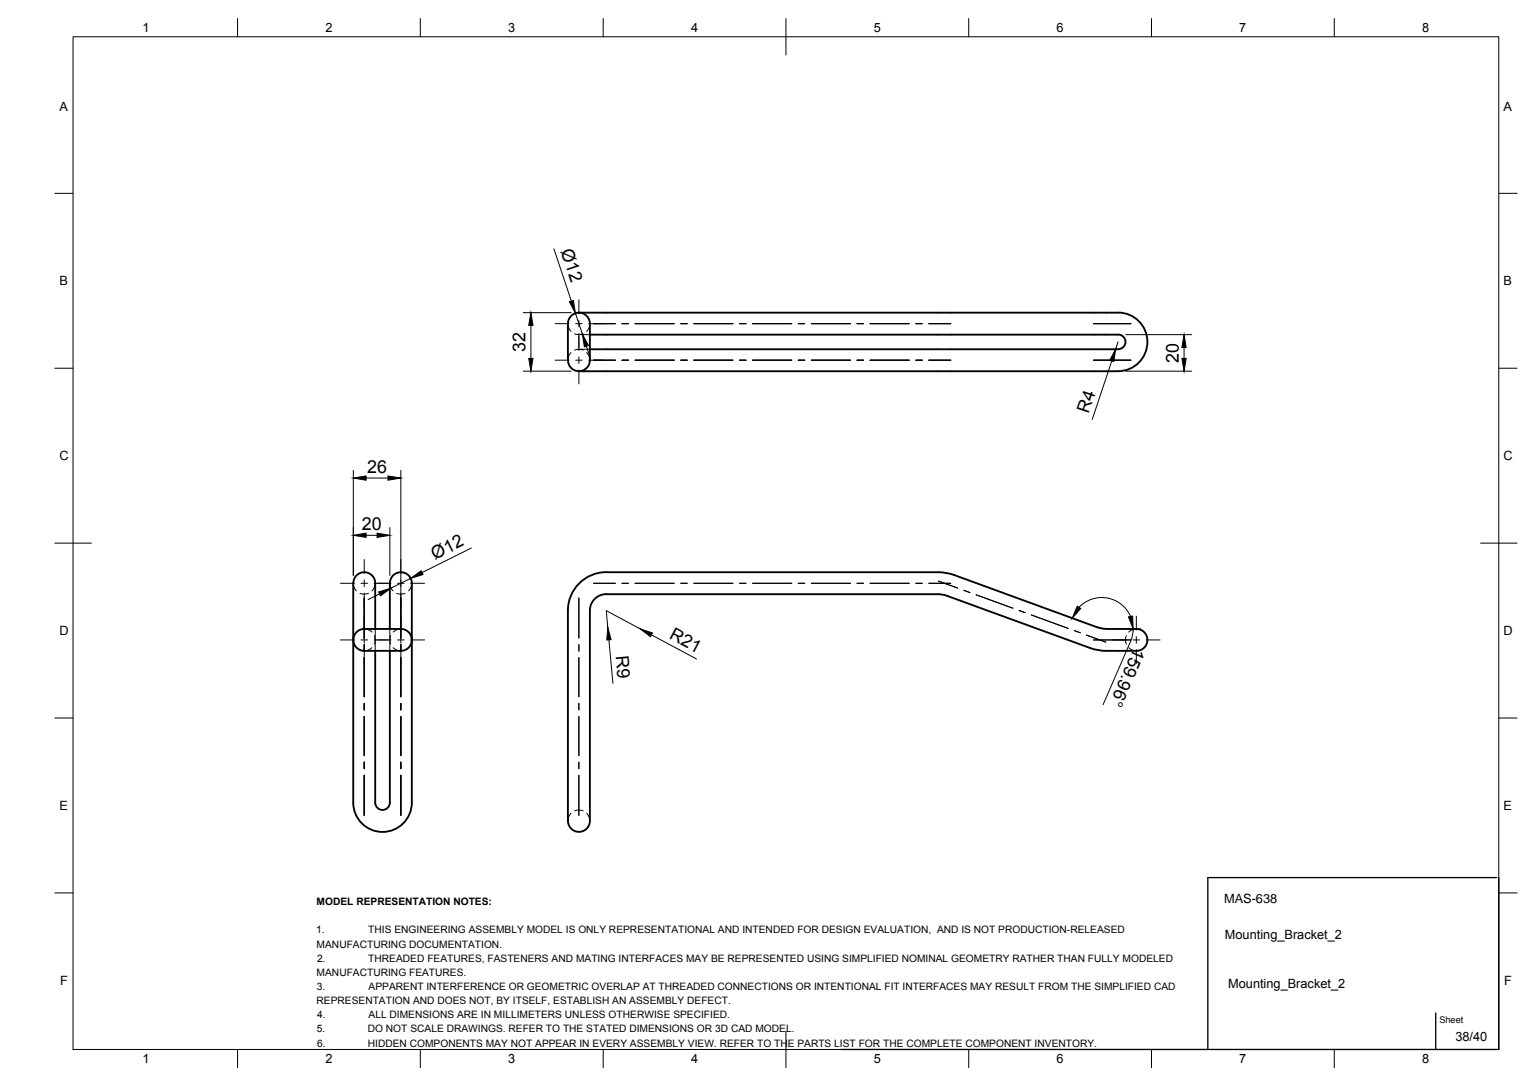
ISO-10303-21;
HEADER;
FILE_DESCRIPTION((''),'2;1');
FILE_NAME('Mounting_Bracket_2.step','2026-10-09T12:00:21-07:00',(''),(''),'','','');
FILE_SCHEMA (('AUTOMOTIVE_DESIGN { 1 0 10303 214 3 1 1 }'));
ENDSEC;
DATA;
#10=MECHANICAL_DESIGN_GEOMETRIC_PRESENTATION_REPRESENTATION('',(#433),#10334);
#168=CYLINDRICAL_SURFACE('',#4326,0.600000000000001) ;
#169=CYLINDRICAL_SURFACE('',#4327,0.600000000000001) ;
#170=CYLINDRICAL_SURFACE('',#4328,0.599999999999996) ;
#171=CYLINDRICAL_SURFACE('',#4329,0.600000000000001) ;
#172=CYLINDRICAL_SURFACE('',#4330,0.600000000000001) ;
#173=CYLINDRICAL_SURFACE('',#4331,0.600000000000001) ;
#174=CYLINDRICAL_SURFACE('',#4332,0.599999999999996) ;
#175=CYLINDRICAL_SURFACE('',#4333,0.600000000000001) ;
#361=SHAPE_REPRESENTATION_RELATIONSHIP('SRR','None',#10479,#393) ;
#393=ADVANCED_BREP_SHAPE_REPRESENTATION('',(#465),#10331) ;
#433=STYLED_ITEM('',(#10631),#465) ;
#465=MANIFOLD_SOLID_BREP('Body1',#3587) ;
#666=LINE('',#10068,#824) ;
#667=LINE('',#10070,#825) ;
#668=LINE('',#10072,#826) ;
#669=LINE('',#10074,#827) ;
#670=LINE('',#10076,#828) ;
#671=LINE('',#10078,#829) ;
#672=LINE('',#10080,#830) ;
#673=LINE('',#10082,#831) ;
#824=VECTOR('',#5346,0.600000000000001) ;
#825=VECTOR('',#5349,0.600000000000001) ;
#826=VECTOR('',#5352,0.599999999999996) ;
#827=VECTOR('',#5355,0.600000000000001) ;
#828=VECTOR('',#5358,0.600000000000001) ;
#829=VECTOR('',#5361,0.600000000000001) ;
#830=VECTOR('',#5364,0.599999999999996) ;
#831=VECTOR('',#5367,0.600000000000001) ;
#1002=FACE_OUTER_BOUND('',#1210,.T.) ;
#1003=FACE_OUTER_BOUND('',#1211,.T.) ;
#1004=FACE_OUTER_BOUND('',#1212,.T.) ;
#1005=FACE_OUTER_BOUND('',#1213,.T.) ;
#1006=FACE_OUTER_BOUND('',#1214,.T.) ;
#1007=FACE_OUTER_BOUND('',#1215,.T.) ;
#1008=FACE_OUTER_BOUND('',#1216,.T.) ;
#1009=FACE_OUTER_BOUND('',#1217,.T.) ;
#1010=FACE_OUTER_BOUND('',#1218,.T.) ;
#1011=FACE_OUTER_BOUND('',#1219,.T.) ;
#1012=FACE_OUTER_BOUND('',#1220,.T.) ;
#1013=FACE_OUTER_BOUND('',#1221,.T.) ;
#1014=FACE_OUTER_BOUND('',#1222,.T.) ;
#1015=FACE_OUTER_BOUND('',#1223,.T.) ;
#1016=FACE_OUTER_BOUND('',#1224,.T.) ;
#1017=FACE_OUTER_BOUND('',#1225,.T.) ;
#1210=EDGE_LOOP('',(#3049,#3050,#3051,#3052,#3053)) ;
#1211=EDGE_LOOP('',(#3054,#3055,#3056,#3057)) ;
#1212=EDGE_LOOP('',(#3058,#3059,#3060,#3061,#3062,#3063)) ;
#1213=EDGE_LOOP('',(#3064,#3065,#3066,#3067,#3068,#3069)) ;
#1214=EDGE_LOOP('',(#3070,#3071,#3072,#3073,#3074,#3075)) ;
#1215=EDGE_LOOP('',(#3076,#3077,#3078,#3079,#3080)) ;
#1216=EDGE_LOOP('',(#3081,#3082,#3083,#3084)) ;
#1217=EDGE_LOOP('',(#3085,#3086,#3087,#3088,#3089,#3090)) ;
#1218=EDGE_LOOP('',(#3091,#3092,#3093,#3094,#3095,#3096)) ;
#1219=EDGE_LOOP('',(#3097,#3098,#3099,#3100)) ;
#1220=EDGE_LOOP('',(#3101,#3102,#3103,#3104,#3105)) ;
#1221=EDGE_LOOP('',(#3106,#3107,#3108,#3109,#3110,#3111)) ;
#1222=EDGE_LOOP('',(#3112,#3113,#3114,#3115,#3116,#3117)) ;
#1223=EDGE_LOOP('',(#3118,#3119,#3120,#3121)) ;
#1224=EDGE_LOOP('',(#3122,#3123,#3124,#3125,#3126)) ;
#1225=EDGE_LOOP('',(#3127,#3128,#3129,#3130,#3131,#3132)) ;
#1397=CIRCLE('',#4285,0.600000000000001) ;
#1398=CIRCLE('',#4286,0.900000000000006) ;
#1399=CIRCLE('',#4287,0.600000000000001) ;
#1400=CIRCLE('',#4288,0.600000000000001) ;
#1401=CIRCLE('',#4290,0.600000000000001) ;
#1402=CIRCLE('',#4291,1.40000000000001) ;
#1403=CIRCLE('',#4292,0.600000000000001) ;
#1404=CIRCLE('',#4294,0.600000000000001) ;
#1405=CIRCLE('',#4295,0.600000000000001) ;
#1406=CIRCLE('',#4296,1.40000000000001) ;
#1407=CIRCLE('',#4297,0.600000000000001) ;
#1408=CIRCLE('',#4298,0.600000000000001) ;
#1409=CIRCLE('',#4300,0.600000000000001) ;
#1410=CIRCLE('',#4301,0.399999999999999) ;
#1411=CIRCLE('',#4302,0.600000000000001) ;
#1412=CIRCLE('',#4303,0.600000000000001) ;
#1413=CIRCLE('',#4304,0.600000000000001) ;
#1414=CIRCLE('',#4306,0.600000000000001) ;
#1415=CIRCLE('',#4307,0.600000000000001) ;
#1416=CIRCLE('',#4308,0.400000000000002) ;
#1417=CIRCLE('',#4309,0.600000000000001) ;
#1418=CIRCLE('',#4310,0.600000000000001) ;
#1419=CIRCLE('',#4312,0.600000000000001) ;
#1420=CIRCLE('',#4313,0.600000000000001) ;
#1421=CIRCLE('',#4314,0.900000000000006) ;
#1422=CIRCLE('',#4315,0.600000000000001) ;
#1423=CIRCLE('',#4317,0.600000000000001) ;
#1424=CIRCLE('',#4318,1.40000000000001) ;
#1425=CIRCLE('',#4319,0.600000000000001) ;
#1426=CIRCLE('',#4321,0.600000000000001) ;
#1427=CIRCLE('',#4322,0.600000000000001) ;
#1428=CIRCLE('',#4323,1.40000000000001) ;
#1429=CIRCLE('',#4324,0.600000000000001) ;
#1430=CIRCLE('',#4325,0.600000000000001) ;
#1732=VERTEX_POINT('',#10000) ;
#1733=VERTEX_POINT('',#10002) ;
#1734=VERTEX_POINT('',#10004) ;
#1735=VERTEX_POINT('',#10008) ;
#1736=VERTEX_POINT('',#10010) ;
#1737=VERTEX_POINT('',#10014) ;
#1738=VERTEX_POINT('',#10015) ;
#1739=VERTEX_POINT('',#10018) ;
#1740=VERTEX_POINT('',#10020) ;
#1741=VERTEX_POINT('',#10024) ;
#1742=VERTEX_POINT('',#10025) ;
#1743=VERTEX_POINT('',#10027) ;
#1744=VERTEX_POINT('',#10029) ;
#1745=VERTEX_POINT('',#10034) ;
#1746=VERTEX_POINT('',#10035) ;
#1747=VERTEX_POINT('',#10038) ;
#1748=VERTEX_POINT('',#10040) ;
#1749=VERTEX_POINT('',#10044) ;
#1750=VERTEX_POINT('',#10045) ;
#1751=VERTEX_POINT('',#10048) ;
#1752=VERTEX_POINT('',#10052) ;
#1753=VERTEX_POINT('',#10054) ;
#1754=VERTEX_POINT('',#10058) ;
#1755=VERTEX_POINT('',#10059) ;
#1756=VERTEX_POINT('',#10062) ;
#1757=VERTEX_POINT('',#10064) ;
#2181=EDGE_CURVE('',#1732,#1732,#1397,.T.) ;
#2182=EDGE_CURVE('',#1732,#1733,#1398,.T.) ;
#2183=EDGE_CURVE('',#1733,#1734,#1399,.T.) ;
#2184=EDGE_CURVE('',#1734,#1733,#1400,.T.) ;
#2185=EDGE_CURVE('',#1735,#1735,#1401,.T.) ;
#2186=EDGE_CURVE('',#1735,#1736,#1402,.T.) ;
#2187=EDGE_CURVE('',#1736,#1736,#1403,.T.) ;
#2188=EDGE_CURVE('',#1737,#1738,#1404,.T.) ;
#2189=EDGE_CURVE('',#1738,#1737,#1405,.T.) ;
#2190=EDGE_CURVE('',#1738,#1739,#1406,.T.) ;
#2191=EDGE_CURVE('',#1739,#1740,#1407,.T.) ;
#2192=EDGE_CURVE('',#1740,#1739,#1408,.T.) ;
#2193=EDGE_CURVE('',#1741,#1742,#1409,.T.) ;
#2194=EDGE_CURVE('',#1742,#1743,#1410,.T.) ;
#2195=EDGE_CURVE('',#1744,#1743,#1411,.T.) ;
#2196=EDGE_CURVE('',#1743,#1744,#1412,.T.) ;
#2197=EDGE_CURVE('',#1742,#1741,#1413,.T.) ;
#2198=EDGE_CURVE('',#1745,#1746,#1414,.T.) ;
#2199=EDGE_CURVE('',#1746,#1745,#1415,.T.) ;
#2200=EDGE_CURVE('',#1746,#1747,#1416,.T.) ;
#2201=EDGE_CURVE('',#1747,#1748,#1417,.T.) ;
#2202=EDGE_CURVE('',#1748,#1747,#1418,.T.) ;
#2203=EDGE_CURVE('',#1749,#1750,#1419,.T.) ;
#2204=EDGE_CURVE('',#1750,#1749,#1420,.T.) ;
#2205=EDGE_CURVE('',#1750,#1751,#1421,.T.) ;
#2206=EDGE_CURVE('',#1751,#1751,#1422,.T.) ;
#2207=EDGE_CURVE('',#1752,#1752,#1423,.T.) ;
#2208=EDGE_CURVE('',#1752,#1753,#1424,.T.) ;
#2209=EDGE_CURVE('',#1753,#1753,#1425,.T.) ;
#2210=EDGE_CURVE('',#1754,#1755,#1426,.T.) ;
#2211=EDGE_CURVE('',#1755,#1754,#1427,.T.) ;
#2212=EDGE_CURVE('',#1755,#1756,#1428,.T.) ;
#2213=EDGE_CURVE('',#1756,#1757,#1429,.T.) ;
#2214=EDGE_CURVE('',#1757,#1756,#1430,.T.) ;
#2215=EDGE_CURVE('',#1745,#1734,#666,.T.) ;
#2216=EDGE_CURVE('',#1732,#1736,#667,.T.) ;
#2217=EDGE_CURVE('',#1735,#1740,#668,.T.) ;
#2218=EDGE_CURVE('',#1737,#1741,#669,.T.) ;
#2219=EDGE_CURVE('',#1748,#1749,#670,.T.) ;
#2220=EDGE_CURVE('',#1751,#1752,#671,.T.) ;
#2221=EDGE_CURVE('',#1753,#1754,#672,.T.) ;
#2222=EDGE_CURVE('',#1757,#1744,#673,.T.) ;
#3049=ORIENTED_EDGE('',*,*,#2181,.F.) ;
#3050=ORIENTED_EDGE('',*,*,#2182,.T.) ;
#3051=ORIENTED_EDGE('',*,*,#2183,.T.) ;
#3052=ORIENTED_EDGE('',*,*,#2184,.T.) ;
#3053=ORIENTED_EDGE('',*,*,#2182,.F.) ;
#3054=ORIENTED_EDGE('',*,*,#2185,.F.) ;
#3055=ORIENTED_EDGE('',*,*,#2186,.T.) ;
#3056=ORIENTED_EDGE('',*,*,#2187,.T.) ;
#3057=ORIENTED_EDGE('',*,*,#2186,.F.) ;
#3058=ORIENTED_EDGE('',*,*,#2188,.F.) ;
#3059=ORIENTED_EDGE('',*,*,#2189,.F.) ;
#3060=ORIENTED_EDGE('',*,*,#2190,.T.) ;
#3061=ORIENTED_EDGE('',*,*,#2191,.T.) ;
#3062=ORIENTED_EDGE('',*,*,#2192,.T.) ;
#3063=ORIENTED_EDGE('',*,*,#2190,.F.) ;
#3064=ORIENTED_EDGE('',*,*,#2193,.T.) ;
#3065=ORIENTED_EDGE('',*,*,#2194,.T.) ;
#3066=ORIENTED_EDGE('',*,*,#2195,.F.) ;
#3067=ORIENTED_EDGE('',*,*,#2196,.F.) ;
#3068=ORIENTED_EDGE('',*,*,#2194,.F.) ;
#3069=ORIENTED_EDGE('',*,*,#2197,.T.) ;
#3070=ORIENTED_EDGE('',*,*,#2198,.F.) ;
#3071=ORIENTED_EDGE('',*,*,#2199,.F.) ;
#3072=ORIENTED_EDGE('',*,*,#2200,.T.) ;
#3073=ORIENTED_EDGE('',*,*,#2201,.T.) ;
#3074=ORIENTED_EDGE('',*,*,#2202,.T.) ;
#3075=ORIENTED_EDGE('',*,*,#2200,.F.) ;
#3076=ORIENTED_EDGE('',*,*,#2203,.F.) ;
#3077=ORIENTED_EDGE('',*,*,#2204,.F.) ;
#3078=ORIENTED_EDGE('',*,*,#2205,.T.) ;
#3079=ORIENTED_EDGE('',*,*,#2206,.T.) ;
#3080=ORIENTED_EDGE('',*,*,#2205,.F.) ;
#3081=ORIENTED_EDGE('',*,*,#2207,.F.) ;
#3082=ORIENTED_EDGE('',*,*,#2208,.T.) ;
#3083=ORIENTED_EDGE('',*,*,#2209,.T.) ;
#3084=ORIENTED_EDGE('',*,*,#2208,.F.) ;
#3085=ORIENTED_EDGE('',*,*,#2210,.F.) ;
#3086=ORIENTED_EDGE('',*,*,#2211,.F.) ;
#3087=ORIENTED_EDGE('',*,*,#2212,.T.) ;
#3088=ORIENTED_EDGE('',*,*,#2213,.T.) ;
#3089=ORIENTED_EDGE('',*,*,#2214,.T.) ;
#3090=ORIENTED_EDGE('',*,*,#2212,.F.) ;
#3091=ORIENTED_EDGE('',*,*,#2198,.T.) ;
#3092=ORIENTED_EDGE('',*,*,#2199,.T.) ;
#3093=ORIENTED_EDGE('',*,*,#2215,.T.) ;
#3094=ORIENTED_EDGE('',*,*,#2183,.F.) ;
#3095=ORIENTED_EDGE('',*,*,#2184,.F.) ;
#3096=ORIENTED_EDGE('',*,*,#2215,.F.) ;
#3097=ORIENTED_EDGE('',*,*,#2181,.T.) ;
#3098=ORIENTED_EDGE('',*,*,#2216,.T.) ;
#3099=ORIENTED_EDGE('',*,*,#2187,.F.) ;
#3100=ORIENTED_EDGE('',*,*,#2216,.F.) ;
#3101=ORIENTED_EDGE('',*,*,#2185,.T.) ;
#3102=ORIENTED_EDGE('',*,*,#2217,.T.) ;
#3103=ORIENTED_EDGE('',*,*,#2191,.F.) ;
#3104=ORIENTED_EDGE('',*,*,#2192,.F.) ;
#3105=ORIENTED_EDGE('',*,*,#2217,.F.) ;
#3106=ORIENTED_EDGE('',*,*,#2188,.T.) ;
#3107=ORIENTED_EDGE('',*,*,#2189,.T.) ;
#3108=ORIENTED_EDGE('',*,*,#2218,.T.) ;
#3109=ORIENTED_EDGE('',*,*,#2197,.F.) ;
#3110=ORIENTED_EDGE('',*,*,#2193,.F.) ;
#3111=ORIENTED_EDGE('',*,*,#2218,.F.) ;
#3112=ORIENTED_EDGE('',*,*,#2202,.F.) ;
#3113=ORIENTED_EDGE('',*,*,#2219,.T.) ;
#3114=ORIENTED_EDGE('',*,*,#2203,.T.) ;
#3115=ORIENTED_EDGE('',*,*,#2204,.T.) ;
#3116=ORIENTED_EDGE('',*,*,#2219,.F.) ;
#3117=ORIENTED_EDGE('',*,*,#2201,.F.) ;
#3118=ORIENTED_EDGE('',*,*,#2206,.F.) ;
#3119=ORIENTED_EDGE('',*,*,#2220,.T.) ;
#3120=ORIENTED_EDGE('',*,*,#2207,.T.) ;
#3121=ORIENTED_EDGE('',*,*,#2220,.F.) ;
#3122=ORIENTED_EDGE('',*,*,#2209,.F.) ;
#3123=ORIENTED_EDGE('',*,*,#2221,.T.) ;
#3124=ORIENTED_EDGE('',*,*,#2210,.T.) ;
#3125=ORIENTED_EDGE('',*,*,#2211,.T.) ;
#3126=ORIENTED_EDGE('',*,*,#2221,.F.) ;
#3127=ORIENTED_EDGE('',*,*,#2214,.F.) ;
#3128=ORIENTED_EDGE('',*,*,#2222,.T.) ;
#3129=ORIENTED_EDGE('',*,*,#2195,.T.) ;
#3130=ORIENTED_EDGE('',*,*,#2196,.T.) ;
#3131=ORIENTED_EDGE('',*,*,#2222,.F.) ;
#3132=ORIENTED_EDGE('',*,*,#2213,.F.) ;
#3335=TOROIDAL_SURFACE('',#4284,1.5,0.6) ;
#3336=TOROIDAL_SURFACE('',#4289,2.,0.6) ;
#3337=TOROIDAL_SURFACE('',#4293,2.,0.6) ;
#3338=TOROIDAL_SURFACE('',#4299,1.,0.6) ;
#3339=TOROIDAL_SURFACE('',#4305,1.,0.599999999999999) ;
#3340=TOROIDAL_SURFACE('',#4311,1.5,0.6) ;
#3341=TOROIDAL_SURFACE('',#4316,2.,0.6) ;
#3342=TOROIDAL_SURFACE('',#4320,2.,0.6) ;
#3510=ADVANCED_FACE('',(#1002),#3335,.T.) ;
#3511=ADVANCED_FACE('',(#1003),#3336,.T.) ;
#3512=ADVANCED_FACE('',(#1004),#3337,.T.) ;
#3513=ADVANCED_FACE('',(#1005),#3338,.T.) ;
#3514=ADVANCED_FACE('',(#1006),#3339,.T.) ;
#3515=ADVANCED_FACE('',(#1007),#3340,.T.) ;
#3516=ADVANCED_FACE('',(#1008),#3341,.T.) ;
#3517=ADVANCED_FACE('',(#1009),#3342,.T.) ;
#3518=ADVANCED_FACE('',(#1010),#168,.T.) ;
#3519=ADVANCED_FACE('',(#1011),#169,.T.) ;
#3520=ADVANCED_FACE('',(#1012),#170,.T.) ;
#3521=ADVANCED_FACE('',(#1013),#171,.T.) ;
#3522=ADVANCED_FACE('',(#1014),#172,.T.) ;
#3523=ADVANCED_FACE('',(#1015),#173,.T.) ;
#3524=ADVANCED_FACE('',(#1016),#174,.T.) ;
#3525=ADVANCED_FACE('',(#1017),#175,.T.) ;
#3587=CLOSED_SHELL('',(#3510,#3511,#3512,#3513,#3514,#3515,#3516,#3517,
#3518,#3519,#3520,#3521,#3522,#3523,#3524,#3525)) ;
#4283=AXIS2_PLACEMENT_3D('',#9998,#5258,#5259) ;
#4284=AXIS2_PLACEMENT_3D('',#9999,#5260,#5261) ;
#4285=AXIS2_PLACEMENT_3D('',#10001,#5262,#5263) ;
#4286=AXIS2_PLACEMENT_3D('',#10003,#5264,#5265) ;
#4287=AXIS2_PLACEMENT_3D('',#10005,#5266,#5267) ;
#4288=AXIS2_PLACEMENT_3D('',#10006,#5268,#5269) ;
#4289=AXIS2_PLACEMENT_3D('',#10007,#5270,#5271) ;
#4290=AXIS2_PLACEMENT_3D('',#10009,#5272,#5273) ;
#4291=AXIS2_PLACEMENT_3D('',#10011,#5274,#5275) ;
#4292=AXIS2_PLACEMENT_3D('',#10012,#5276,#5277) ;
#4293=AXIS2_PLACEMENT_3D('',#10013,#5278,#5279) ;
#4294=AXIS2_PLACEMENT_3D('',#10016,#5280,#5281) ;
#4295=AXIS2_PLACEMENT_3D('',#10017,#5282,#5283) ;
#4296=AXIS2_PLACEMENT_3D('',#10019,#5284,#5285) ;
#4297=AXIS2_PLACEMENT_3D('',#10021,#5286,#5287) ;
#4298=AXIS2_PLACEMENT_3D('',#10022,#5288,#5289) ;
#4299=AXIS2_PLACEMENT_3D('',#10023,#5290,#5291) ;
#4300=AXIS2_PLACEMENT_3D('',#10026,#5292,#5293) ;
#4301=AXIS2_PLACEMENT_3D('',#10028,#5294,#5295) ;
#4302=AXIS2_PLACEMENT_3D('',#10030,#5296,#5297) ;
#4303=AXIS2_PLACEMENT_3D('',#10031,#5298,#5299) ;
#4304=AXIS2_PLACEMENT_3D('',#10032,#5300,#5301) ;
#4305=AXIS2_PLACEMENT_3D('',#10033,#5302,#5303) ;
#4306=AXIS2_PLACEMENT_3D('',#10036,#5304,#5305) ;
#4307=AXIS2_PLACEMENT_3D('',#10037,#5306,#5307) ;
#4308=AXIS2_PLACEMENT_3D('',#10039,#5308,#5309) ;
#4309=AXIS2_PLACEMENT_3D('',#10041,#5310,#5311) ;
#4310=AXIS2_PLACEMENT_3D('',#10042,#5312,#5313) ;
#4311=AXIS2_PLACEMENT_3D('',#10043,#5314,#5315) ;
#4312=AXIS2_PLACEMENT_3D('',#10046,#5316,#5317) ;
#4313=AXIS2_PLACEMENT_3D('',#10047,#5318,#5319) ;
#4314=AXIS2_PLACEMENT_3D('',#10049,#5320,#5321) ;
#4315=AXIS2_PLACEMENT_3D('',#10050,#5322,#5323) ;
#4316=AXIS2_PLACEMENT_3D('',#10051,#5324,#5325) ;
#4317=AXIS2_PLACEMENT_3D('',#10053,#5326,#5327) ;
#4318=AXIS2_PLACEMENT_3D('',#10055,#5328,#5329) ;
#4319=AXIS2_PLACEMENT_3D('',#10056,#5330,#5331) ;
#4320=AXIS2_PLACEMENT_3D('',#10057,#5332,#5333) ;
#4321=AXIS2_PLACEMENT_3D('',#10060,#5334,#5335) ;
#4322=AXIS2_PLACEMENT_3D('',#10061,#5336,#5337) ;
#4323=AXIS2_PLACEMENT_3D('',#10063,#5338,#5339) ;
#4324=AXIS2_PLACEMENT_3D('',#10065,#5340,#5341) ;
#4325=AXIS2_PLACEMENT_3D('',#10066,#5342,#5343) ;
#4326=AXIS2_PLACEMENT_3D('',#10067,#5344,#5345) ;
#4327=AXIS2_PLACEMENT_3D('',#10069,#5347,#5348) ;
#4328=AXIS2_PLACEMENT_3D('',#10071,#5350,#5351) ;
#4329=AXIS2_PLACEMENT_3D('',#10073,#5353,#5354) ;
#4330=AXIS2_PLACEMENT_3D('',#10075,#5356,#5357) ;
#4331=AXIS2_PLACEMENT_3D('',#10077,#5359,#5360) ;
#4332=AXIS2_PLACEMENT_3D('',#10079,#5362,#5363) ;
#4333=AXIS2_PLACEMENT_3D('',#10081,#5365,#5366) ;
#5258=DIRECTION('axis',(0.,0.,1.)) ;
#5259=DIRECTION('refdir',(1.,0.,0.)) ;
#5260=DIRECTION('center_axis',(-1.,0.,-3.38946600347724E-15)) ;
#5261=DIRECTION('ref_axis',(3.38353683695287E-15,0.,-1.)) ;
#5262=DIRECTION('center_axis',(3.38946600347724E-15,0.,-1.)) ;
#5263=DIRECTION('ref_axis',(-1.,0.,-3.38946600347724E-15)) ;
#5264=DIRECTION('center_axis',(1.,0.,3.38946600347724E-15)) ;
#5265=DIRECTION('ref_axis',(3.38946600347724E-15,0.,-1.)) ;
#5266=DIRECTION('center_axis',(0.,1.,0.)) ;
#5267=DIRECTION('ref_axis',(-1.,0.,0.)) ;
#5268=DIRECTION('center_axis',(0.,1.,0.)) ;
#5269=DIRECTION('ref_axis',(-1.,0.,0.)) ;
#5270=DIRECTION('center_axis',(-1.,0.,-3.38946600347724E-15)) ;
#5271=DIRECTION('ref_axis',(4.09928501400059E-15,0.,-1.)) ;
#5272=DIRECTION('center_axis',(3.1843026467959E-15,-0.342630345100702,-0.93947030108257)) ;
#5273=DIRECTION('ref_axis',(-1.,-1.09103871477676E-15,-2.99155776632337E-15)) ;
#5274=DIRECTION('center_axis',(1.,0.,3.38946600347724E-15)) ;
#5275=DIRECTION('ref_axis',(3.38946600347724E-15,0.,-1.)) ;
#5276=DIRECTION('center_axis',(3.38946600347724E-15,0.,-1.)) ;
#5277=DIRECTION('ref_axis',(-1.,0.,-3.38946600347724E-15)) ;
#5278=DIRECTION('center_axis',(1.,0.,3.38946600347724E-15)) ;
#5279=DIRECTION('ref_axis',(-4.09928501400059E-15,0.,1.)) ;
#5280=DIRECTION('center_axis',(3.38946600347724E-15,0.,-1.)) ;
#5281=DIRECTION('ref_axis',(-1.,0.,-3.38946600347724E-15)) ;
#5282=DIRECTION('center_axis',(3.38946600347724E-15,0.,-1.)) ;
#5283=DIRECTION('ref_axis',(-1.,0.,-3.38946600347724E-15)) ;
#5284=DIRECTION('center_axis',(-1.,0.,-3.38946600347724E-15)) ;
#5285=DIRECTION('ref_axis',(-3.38946600347724E-15,0.,1.)) ;
#5286=DIRECTION('center_axis',(3.1843026467959E-15,-0.342630345100702,-0.93947030108257)) ;
#5287=DIRECTION('ref_axis',(-1.,-1.09103871477676E-15,-2.99155776632337E-15)) ;
#5288=DIRECTION('center_axis',(3.1843026467959E-15,-0.342630345100702,-0.93947030108257)) ;
#5289=DIRECTION('ref_axis',(-1.,-1.09103871477676E-15,-2.99155776632337E-15)) ;
#5290=DIRECTION('center_axis',(0.,-1.,0.)) ;
#5291=DIRECTION('ref_axis',(1.,0.,0.)) ;
#5292=DIRECTION('center_axis',(3.38946600347724E-15,0.,-1.)) ;
#5293=DIRECTION('ref_axis',(-1.,0.,-3.38946600347724E-15)) ;
#5294=DIRECTION('center_axis',(0.,1.,0.)) ;
#5295=DIRECTION('ref_axis',(1.,0.,0.)) ;
#5296=DIRECTION('center_axis',(-3.49148133884313E-15,0.,1.)) ;
#5297=DIRECTION('ref_axis',(1.,0.,3.49148133884313E-15)) ;
#5298=DIRECTION('center_axis',(-3.49148133884313E-15,0.,1.)) ;
#5299=DIRECTION('ref_axis',(1.,0.,3.49148133884313E-15)) ;
#5300=DIRECTION('center_axis',(3.38946600347724E-15,0.,-1.)) ;
#5301=DIRECTION('ref_axis',(-1.,0.,-3.38946600347724E-15)) ;
#5302=DIRECTION('center_axis',(-3.49148133884313E-15,0.,1.)) ;
#5303=DIRECTION('ref_axis',(1.,0.,0.)) ;
#5304=DIRECTION('center_axis',(0.,1.,0.)) ;
#5305=DIRECTION('ref_axis',(-1.,0.,0.)) ;
#5306=DIRECTION('center_axis',(0.,1.,0.)) ;
#5307=DIRECTION('ref_axis',(-1.,0.,0.)) ;
#5308=DIRECTION('center_axis',(3.49148133884313E-15,0.,-1.)) ;
#5309=DIRECTION('ref_axis',(1.,0.,3.49148133884313E-15)) ;
#5310=DIRECTION('center_axis',(0.,-1.,0.)) ;
#5311=DIRECTION('ref_axis',(1.,0.,0.)) ;
#5312=DIRECTION('center_axis',(0.,-1.,0.)) ;
#5313=DIRECTION('ref_axis',(1.,0.,0.)) ;
#5314=DIRECTION('center_axis',(1.,0.,3.49148133884313E-15)) ;
#5315=DIRECTION('ref_axis',(3.38353683695287E-15,0.,-1.)) ;
#5316=DIRECTION('center_axis',(0.,-1.,0.)) ;
#5317=DIRECTION('ref_axis',(1.,0.,0.)) ;
#5318=DIRECTION('center_axis',(0.,-1.,0.)) ;
#5319=DIRECTION('ref_axis',(1.,0.,0.)) ;
#5320=DIRECTION('center_axis',(-1.,0.,-3.49148133884313E-15)) ;
#5321=DIRECTION('ref_axis',(3.49148133884313E-15,0.,-1.)) ;
#5322=DIRECTION('center_axis',(-3.49148133884313E-15,0.,1.)) ;
#5323=DIRECTION('ref_axis',(1.,0.,3.49148133884313E-15)) ;
#5324=DIRECTION('center_axis',(1.,0.,3.49148133884313E-15)) ;
#5325=DIRECTION('ref_axis',(4.09928501400059E-15,0.,-1.)) ;
#5326=DIRECTION('center_axis',(-3.49148133884313E-15,0.,1.)) ;
#5327=DIRECTION('ref_axis',(1.,0.,3.49148133884313E-15)) ;
#5328=DIRECTION('center_axis',(-1.,0.,-3.49148133884313E-15)) ;
#5329=DIRECTION('ref_axis',(3.49148133884313E-15,0.,-1.)) ;
#5330=DIRECTION('center_axis',(-3.28014302462713E-15,0.342630345100702,
0.93947030108257)) ;
#5331=DIRECTION('ref_axis',(1.,1.12387653650765E-15,3.08159695494034E-15)) ;
#5332=DIRECTION('center_axis',(-1.,0.,-3.49148133884313E-15)) ;
#5333=DIRECTION('ref_axis',(-4.09928501400059E-15,0.,1.)) ;
#5334=DIRECTION('center_axis',(-3.28014302462713E-15,0.342630345100702,
0.93947030108257)) ;
#5335=DIRECTION('ref_axis',(1.,1.12387653650765E-15,3.08159695494034E-15)) ;
#5336=DIRECTION('center_axis',(-3.28014302462713E-15,0.342630345100702,
0.93947030108257)) ;
#5337=DIRECTION('ref_axis',(1.,1.12387653650765E-15,3.08159695494034E-15)) ;
#5338=DIRECTION('center_axis',(1.,0.,3.49148133884313E-15)) ;
#5339=DIRECTION('ref_axis',(-3.49148133884313E-15,0.,1.)) ;
#5340=DIRECTION('center_axis',(-3.49148133884313E-15,0.,1.)) ;
#5341=DIRECTION('ref_axis',(1.,0.,3.49148133884313E-15)) ;
#5342=DIRECTION('center_axis',(-3.49148133884313E-15,0.,1.)) ;
#5343=DIRECTION('ref_axis',(1.,0.,3.49148133884313E-15)) ;
#5344=DIRECTION('center_axis',(0.,-1.,0.)) ;
#5345=DIRECTION('ref_axis',(-1.,0.,0.)) ;
#5346=DIRECTION('',(0.,1.,0.)) ;
#5347=DIRECTION('center_axis',(-3.38946600347724E-15,1.91189112624469E-17,
1.)) ;
#5348=DIRECTION('ref_axis',(6.48028997475618E-32,1.,-1.91189112624469E-17)) ;
#5349=DIRECTION('',(3.38946600347724E-15,-1.91189112624469E-17,-1.)) ;
#5350=DIRECTION('center_axis',(-3.1843026467959E-15,0.342630345100702,0.93947030108257)) ;
#5351=DIRECTION('ref_axis',(1.13665102922496E-30,0.93947030108257,-0.342630345100702)) ;
#5352=DIRECTION('',(3.1843026467959E-15,-0.342630345100702,-0.93947030108257)) ;
#5353=DIRECTION('center_axis',(-3.38946600347724E-15,0.,1.)) ;
#5354=DIRECTION('ref_axis',(-1.,0.,-3.38946600347724E-15)) ;
#5355=DIRECTION('',(3.38946600347724E-15,0.,-1.)) ;
#5356=DIRECTION('center_axis',(0.,-1.,0.)) ;
#5357=DIRECTION('ref_axis',(1.,0.,0.)) ;
#5358=DIRECTION('',(0.,1.,0.)) ;
#5359=DIRECTION('center_axis',(-3.49148133884313E-15,1.91189112624469E-17,
1.)) ;
#5360=DIRECTION('ref_axis',(6.6753321891831E-32,1.,-1.91189112624469E-17)) ;
#5361=DIRECTION('',(3.49148133884313E-15,-1.91189112624469E-17,-1.)) ;
#5362=DIRECTION('center_axis',(-3.28014302462713E-15,0.342630345100702,
0.93947030108257)) ;
#5363=DIRECTION('ref_axis',(1.24553608015764E-30,0.93947030108257,-0.342630345100702)) ;
#5364=DIRECTION('',(3.28014302462713E-15,-0.342630345100702,-0.93947030108257)) ;
#5365=DIRECTION('center_axis',(-3.49148133884313E-15,0.,1.)) ;
#5366=DIRECTION('ref_axis',(1.,0.,3.49148133884313E-15)) ;
#5367=DIRECTION('',(3.49148133884313E-15,0.,-1.)) ;
#9998=CARTESIAN_POINT('',(0.,0.,0.)) ;
#9999=CARTESIAN_POINT('Origin',(24.4776880157598,67.0830586252741,103.472433740002)) ;
#10000=CARTESIAN_POINT('',(24.4776880157598,67.9830586252741,103.472433740002)) ;
#10001=CARTESIAN_POINT('Origin',(24.4776880157598,68.5830586252741,103.472433740002)) ;
#10002=CARTESIAN_POINT('',(24.4776880157598,67.0830586252741,104.372433740002)) ;
#10003=CARTESIAN_POINT('Origin',(24.4776880157598,67.0830586252741,103.472433740002)) ;
#10004=CARTESIAN_POINT('',(25.0776880157598,67.0830586252741,104.972433740002)) ;
#10005=CARTESIAN_POINT('Origin',(24.4776880157598,67.0830586252741,104.972433740002)) ;
#10006=CARTESIAN_POINT('Origin',(24.4776880157598,67.0830586252741,104.972433740002)) ;
#10007=CARTESIAN_POINT('Origin',(24.4776880157599,66.5830586252741,85.3257573716235)) ;
#10008=CARTESIAN_POINT('',(24.4776880157599,67.8983170467897,84.8460748884825)) ;
#10009=CARTESIAN_POINT('Origin',(24.4776880157599,68.4619992274392,84.6404966814221)) ;
#10010=CARTESIAN_POINT('',(24.4776880157598,67.9830586252741,85.3257573716235)) ;
#10011=CARTESIAN_POINT('Origin',(24.4776880157599,66.5830586252741,85.3257573716235)) ;
#10012=CARTESIAN_POINT('Origin',(24.4776880157599,68.5830586252741,85.3257573716235)) ;
#10013=CARTESIAN_POINT('Origin',(24.4776880157599,67.4830586252741,76.1191101083796)) ;
#10014=CARTESIAN_POINT('',(25.0776880157599,65.4830586252741,76.1191101083796)) ;
#10015=CARTESIAN_POINT('',(24.4776880157599,66.0830586252741,76.1191101083796)) ;
#10016=CARTESIAN_POINT('Origin',(24.4776880157599,65.4830586252741,76.1191101083796)) ;
#10017=CARTESIAN_POINT('Origin',(24.4776880157599,65.4830586252741,76.1191101083796)) ;
#10018=CARTESIAN_POINT('',(24.4776880157599,66.1678002037585,76.5987925915206)) ;
#10019=CARTESIAN_POINT('Origin',(24.4776880157599,67.4830586252741,76.1191101083796)) ;
#10020=CARTESIAN_POINT('',(24.4776880157599,65.0404358424594,77.0099490056414)) ;
#10021=CARTESIAN_POINT('Origin',(24.4776880157599,65.604118023109,76.804370798581)) ;
#10022=CARTESIAN_POINT('Origin',(24.4776880157599,65.604118023109,76.804370798581)) ;
#10023=CARTESIAN_POINT('Origin',(23.4776880157599,65.4830586252741,75.4724337400015)) ;
#10024=CARTESIAN_POINT('',(25.0776880157599,65.4830586252741,75.4724337400016)) ;
#10025=CARTESIAN_POINT('',(23.8776880157599,65.4830586252741,75.4724337400016)) ;
#10026=CARTESIAN_POINT('Origin',(24.4776880157599,65.4830586252741,75.4724337400016)) ;
#10027=CARTESIAN_POINT('',(23.0776880157599,65.4830586252741,75.4724337400015)) ;
#10028=CARTESIAN_POINT('Origin',(23.4776880157599,65.4830586252741,75.4724337400015)) ;
#10029=CARTESIAN_POINT('',(21.8776880157599,65.4830586252741,75.4724337400015)) ;
#10030=CARTESIAN_POINT('Origin',(22.4776880157599,65.4830586252741,75.4724337400015)) ;
#10031=CARTESIAN_POINT('Origin',(22.4776880157599,65.4830586252741,75.4724337400015)) ;
#10032=CARTESIAN_POINT('Origin',(24.4776880157599,65.4830586252741,75.4724337400016)) ;
#10033=CARTESIAN_POINT('Origin',(23.4776880157598,56.5830586252741,104.972433740002)) ;
#10034=CARTESIAN_POINT('',(25.0776880157598,56.5830586252741,104.972433740002)) ;
#10035=CARTESIAN_POINT('',(23.8776880157598,56.5830586252741,104.972433740002)) ;
#10036=CARTESIAN_POINT('Origin',(24.4776880157598,56.5830586252741,104.972433740002)) ;
#10037=CARTESIAN_POINT('Origin',(24.4776880157598,56.5830586252741,104.972433740002)) ;
#10038=CARTESIAN_POINT('',(23.0776880157598,56.5830586252741,104.972433740002)) ;
#10039=CARTESIAN_POINT('Origin',(23.4776880157598,56.5830586252741,104.972433740002)) ;
#10040=CARTESIAN_POINT('',(21.8776880157598,56.5830586252741,104.972433740002)) ;
#10041=CARTESIAN_POINT('Origin',(22.4776880157598,56.5830586252741,104.972433740002)) ;
#10042=CARTESIAN_POINT('Origin',(22.4776880157598,56.5830586252741,104.972433740002)) ;
#10043=CARTESIAN_POINT('Origin',(22.4776880157598,67.0830586252741,103.472433740002)) ;
#10044=CARTESIAN_POINT('',(21.8776880157598,67.0830586252741,104.972433740002)) ;
#10045=CARTESIAN_POINT('',(22.4776880157598,67.0830586252741,104.372433740002)) ;
#10046=CARTESIAN_POINT('Origin',(22.4776880157598,67.0830586252741,104.972433740002)) ;
#10047=CARTESIAN_POINT('Origin',(22.4776880157598,67.0830586252741,104.972433740002)) ;
#10048=CARTESIAN_POINT('',(22.4776880157598,67.9830586252741,103.472433740002)) ;
#10049=CARTESIAN_POINT('Origin',(22.4776880157598,67.0830586252741,103.472433740002)) ;
#10050=CARTESIAN_POINT('Origin',(22.4776880157598,68.5830586252741,103.472433740002)) ;
#10051=CARTESIAN_POINT('Origin',(22.4776880157599,66.5830586252741,85.3257573716235)) ;
#10052=CARTESIAN_POINT('',(22.4776880157598,67.9830586252741,85.3257573716235)) ;
#10053=CARTESIAN_POINT('Origin',(22.4776880157599,68.5830586252741,85.3257573716235)) ;
#10054=CARTESIAN_POINT('',(22.4776880157599,67.8983170467897,84.8460748884825)) ;
#10055=CARTESIAN_POINT('Origin',(22.4776880157599,66.5830586252741,85.3257573716235)) ;
#10056=CARTESIAN_POINT('Origin',(22.4776880157599,68.4619992274392,84.6404966814221)) ;
#10057=CARTESIAN_POINT('Origin',(22.4776880157599,67.4830586252741,76.1191101083796)) ;
#10058=CARTESIAN_POINT('',(22.4776880157599,65.0404358424594,77.0099490056414)) ;
#10059=CARTESIAN_POINT('',(22.4776880157599,66.1678002037585,76.5987925915206)) ;
#10060=CARTESIAN_POINT('Origin',(22.4776880157599,65.604118023109,76.804370798581)) ;
#10061=CARTESIAN_POINT('Origin',(22.4776880157599,65.604118023109,76.804370798581)) ;
#10062=CARTESIAN_POINT('',(22.4776880157599,66.0830586252741,76.1191101083796)) ;
#10063=CARTESIAN_POINT('Origin',(22.4776880157599,67.4830586252741,76.1191101083796)) ;
#10064=CARTESIAN_POINT('',(21.8776880157599,65.4830586252741,76.1191101083796)) ;
#10065=CARTESIAN_POINT('Origin',(22.4776880157599,65.4830586252741,76.1191101083796)) ;
#10066=CARTESIAN_POINT('Origin',(22.4776880157599,65.4830586252741,76.1191101083796)) ;
#10067=CARTESIAN_POINT('Origin',(24.4776880157598,67.0830586252741,104.972433740002)) ;
#10068=CARTESIAN_POINT('',(25.0776880157598,67.0830586252741,104.972433740002)) ;
#10069=CARTESIAN_POINT('Origin',(24.4776880157599,68.5830586252741,85.3257573716235)) ;
#10070=CARTESIAN_POINT('',(24.4776880157599,67.9830586252741,85.3257573716235)) ;
#10071=CARTESIAN_POINT('Origin',(24.4776880157599,65.6041180231089,76.804370798581)) ;
#10072=CARTESIAN_POINT('',(24.4776880157599,65.0404358424594,77.0099490056414)) ;
#10073=CARTESIAN_POINT('Origin',(24.4776880157599,65.4830586252741,75.4724337400016)) ;
#10074=CARTESIAN_POINT('',(25.0776880157599,65.4830586252741,75.4724337400016)) ;
#10075=CARTESIAN_POINT('Origin',(22.4776880157598,67.0830586252741,104.972433740002)) ;
#10076=CARTESIAN_POINT('',(21.8776880157598,67.0830586252741,104.972433740002)) ;
#10077=CARTESIAN_POINT('Origin',(22.4776880157599,68.5830586252741,85.3257573716235)) ;
#10078=CARTESIAN_POINT('',(22.4776880157599,67.9830586252741,85.3257573716235)) ;
#10079=CARTESIAN_POINT('Origin',(22.4776880157599,65.6041180231089,76.804370798581)) ;
#10080=CARTESIAN_POINT('',(22.4776880157599,65.0404358424594,77.0099490056414)) ;
#10081=CARTESIAN_POINT('Origin',(22.4776880157599,65.4830586252741,75.4724337400015)) ;
#10082=CARTESIAN_POINT('',(21.8776880157599,65.4830586252741,75.4724337400015)) ;
#10294=UNCERTAINTY_MEASURE_WITH_UNIT(LENGTH_MEASURE(0.001),#10335,
'DISTANCE_ACCURACY_VALUE',
'Maximum model space distance between geometric entities at asserted c
onnectivities') ;
#10297=UNCERTAINTY_MEASURE_WITH_UNIT(LENGTH_MEASURE(0.001),#10335,
'DISTANCE_ACCURACY_VALUE',
'Maximum model space distance between geometric entities at asserted c
onnectivities') ;
#10331=(
GEOMETRIC_REPRESENTATION_CONTEXT(3)
GLOBAL_UNCERTAINTY_ASSIGNED_CONTEXT((#10294))
GLOBAL_UNIT_ASSIGNED_CONTEXT((#10335,#10337,#10338))
REPRESENTATION_CONTEXT('','3D')
) ;
#10334=(
GEOMETRIC_REPRESENTATION_CONTEXT(3)
GLOBAL_UNCERTAINTY_ASSIGNED_CONTEXT((#10297))
GLOBAL_UNIT_ASSIGNED_CONTEXT((#10335,#10337,#10338))
REPRESENTATION_CONTEXT('','3D')
) ;
#10335=(
LENGTH_UNIT()
NAMED_UNIT(*)
SI_UNIT(.CENTI.,.METRE.)
) ;
#10337=(
NAMED_UNIT(*)
PLANE_ANGLE_UNIT()
SI_UNIT($,.RADIAN.)
) ;
#10338=(
NAMED_UNIT(*)
SI_UNIT($,.STERADIAN.)
SOLID_ANGLE_UNIT()
) ;
#10372=SHAPE_DEFINITION_REPRESENTATION(#10435,#10479) ;
#10435=PRODUCT_DEFINITION_SHAPE('',$,#10516) ;
#10479=SHAPE_REPRESENTATION('',(#4283),#10331) ;
#10482=PRODUCT_DEFINITION_CONTEXT('part definition',#10592,'design') ;
#10516=PRODUCT_DEFINITION('Mounting_Bracket_2','Mounting_Bracket_2',#10552,
#10482) ;
#10552=PRODUCT_DEFINITION_FORMATION('',$,#10627) ;
#10592=APPLICATION_CONTEXT(
'Core Data for Automotive Mechanical Design Process') ;
#10593=PRODUCT_CONTEXT('part definition',#10592,'mechanical') ;
#10627=PRODUCT('Mounting_Bracket_2','Mounting_Bracket_2',$,(#10593)) ;
#10631=PRESENTATION_STYLE_ASSIGNMENT((#10635)) ;
#10635=SURFACE_STYLE_USAGE(.BOTH.,#10639) ;
#10639=SURFACE_SIDE_STYLE('',(#10643)) ;
#10643=SURFACE_STYLE_FILL_AREA(#10647) ;
#10647=FILL_AREA_STYLE('Opaque(25,25,25)',(#10651)) ;
#10651=FILL_AREA_STYLE_COLOUR('Opaque(25,25,25)',#10655) ;
#10655=COLOUR_RGB('Opaque(25,25,25)', 0.09019608, 0.27058824, 0.51372549) ;
ENDSEC;
END-ISO-10303-21;
